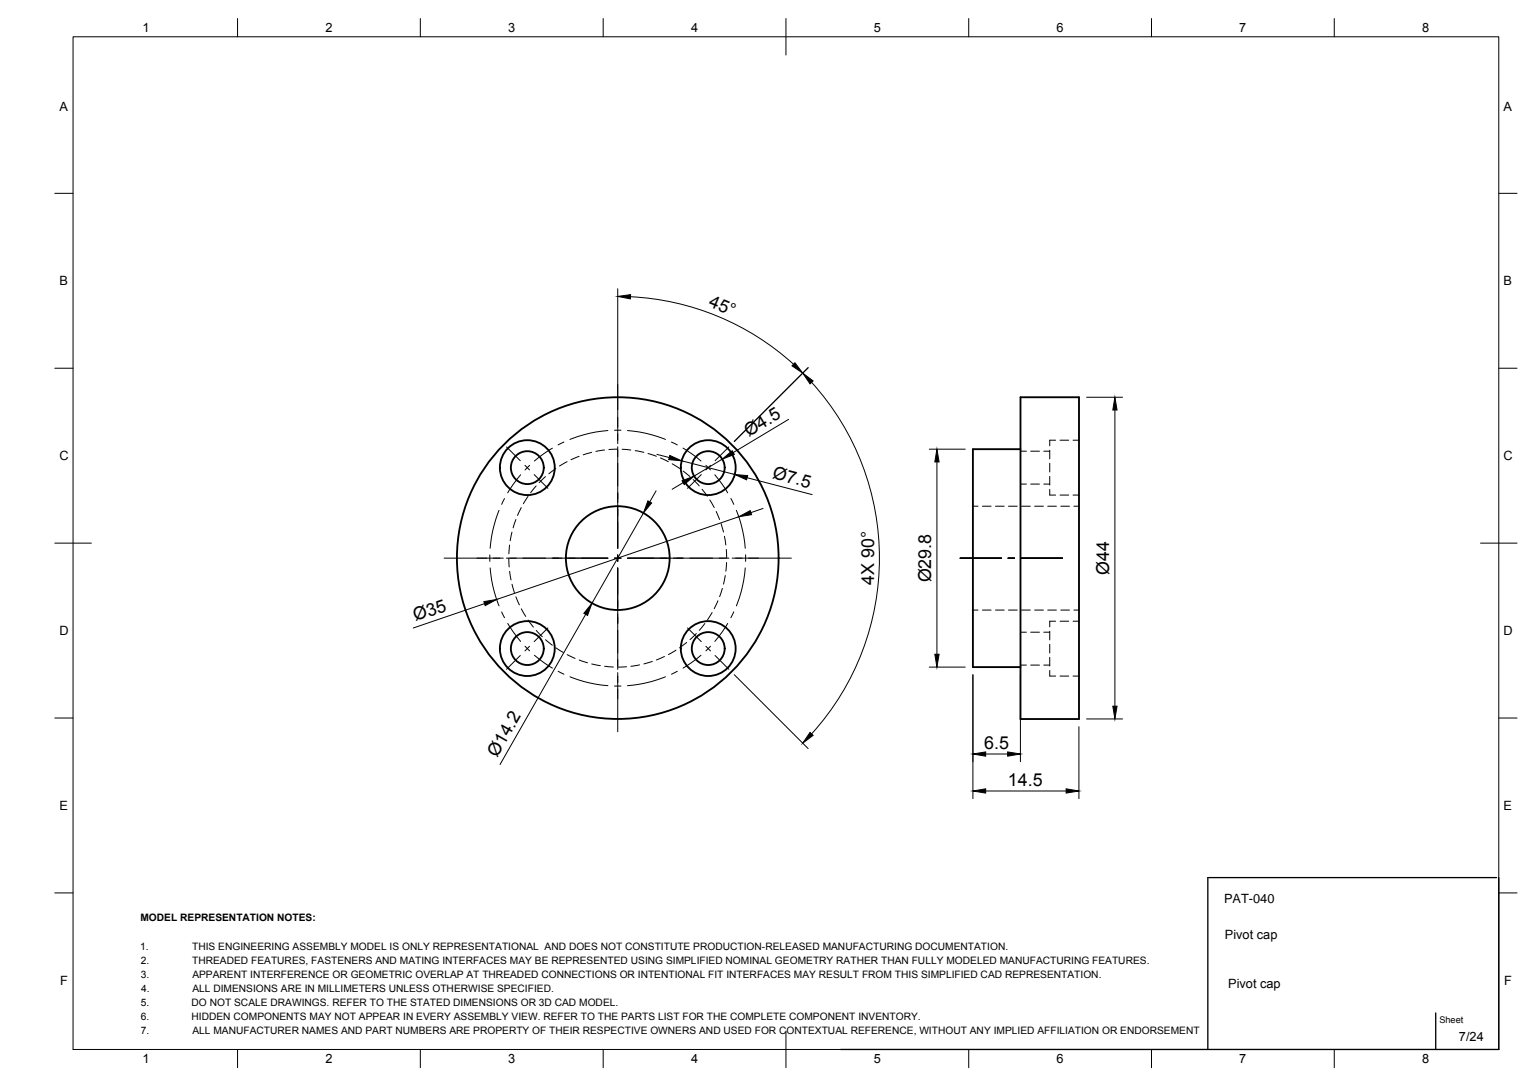
ISO-10303-21;
HEADER;
/* Generated by software containing ST-Developer
 * from STEP Tools, Inc. (www.steptools.com) 
 */

FILE_DESCRIPTION(
/* description */ ('Four-bar tabletop demonstrator'),
/* implementation_level */ '2;1');

FILE_NAME(
/* name */ 'Pivot cap.step',
/* time_stamp */ '2026-10-29T17:05:23-07:00',
/* author */ (''),
/* organization */ (''),
/* preprocessor_version */ 'ST-DEVELOPER v20.2',
/* originating_system */ 'Autodesk Translation Framework v15.17.0.0',
/* authorisation */ '');

FILE_SCHEMA (('AUTOMOTIVE_DESIGN { 1 0 10303 214 3 1 1 }'));
ENDSEC;

DATA;
#10=MECHANICAL_DESIGN_GEOMETRIC_PRESENTATION_REPRESENTATION('',(#354),#6705);
#316=SHAPE_REPRESENTATION_RELATIONSHIP('SRR','None',#6825,#331);
#331=ADVANCED_BREP_SHAPE_REPRESENTATION('',(#376),#6698);
#354=STYLED_ITEM('',(#6975),#376);
#376=MANIFOLD_SOLID_BREP('Body1',#3399);
#435=FACE_BOUND('',#954,.T.);
#436=FACE_BOUND('',#957,.T.);
#437=FACE_BOUND('',#960,.T.);
#438=FACE_BOUND('',#963,.T.);
#439=FACE_BOUND('',#970,.T.);
#440=FACE_BOUND('',#974,.T.);
#441=FACE_BOUND('',#975,.T.);
#442=FACE_BOUND('',#976,.T.);
#443=FACE_BOUND('',#977,.T.);
#444=FACE_BOUND('',#978,.T.);
#445=FACE_BOUND('',#980,.T.);
#446=FACE_BOUND('',#981,.T.);
#447=FACE_BOUND('',#982,.T.);
#448=FACE_BOUND('',#983,.T.);
#449=FACE_BOUND('',#984,.T.);
#521=PLANE('',#3885);
#522=PLANE('',#3890);
#523=PLANE('',#3895);
#524=PLANE('',#3900);
#525=PLANE('',#3913);
#526=PLANE('',#3920);
#527=PLANE('',#3921);
#695=FACE_OUTER_BOUND('',#952,.T.);
#696=FACE_OUTER_BOUND('',#953,.T.);
#697=FACE_OUTER_BOUND('',#955,.T.);
#698=FACE_OUTER_BOUND('',#956,.T.);
#699=FACE_OUTER_BOUND('',#958,.T.);
#700=FACE_OUTER_BOUND('',#959,.T.);
#701=FACE_OUTER_BOUND('',#961,.T.);
#702=FACE_OUTER_BOUND('',#962,.T.);
#703=FACE_OUTER_BOUND('',#964,.T.);
#704=FACE_OUTER_BOUND('',#965,.T.);
#705=FACE_OUTER_BOUND('',#966,.T.);
#706=FACE_OUTER_BOUND('',#967,.T.);
#707=FACE_OUTER_BOUND('',#968,.T.);
#708=FACE_OUTER_BOUND('',#969,.T.);
#709=FACE_OUTER_BOUND('',#971,.T.);
#710=FACE_OUTER_BOUND('',#972,.T.);
#711=FACE_OUTER_BOUND('',#973,.T.);
#712=FACE_OUTER_BOUND('',#979,.T.);
#952=EDGE_LOOP('',(#2840,#2841,#2842,#2843));
#953=EDGE_LOOP('',(#2844));
#954=EDGE_LOOP('',(#2845));
#955=EDGE_LOOP('',(#2846,#2847,#2848,#2849));
#956=EDGE_LOOP('',(#2850));
#957=EDGE_LOOP('',(#2851));
#958=EDGE_LOOP('',(#2852,#2853,#2854,#2855));
#959=EDGE_LOOP('',(#2856));
#960=EDGE_LOOP('',(#2857));
#961=EDGE_LOOP('',(#2858,#2859,#2860,#2861));
#962=EDGE_LOOP('',(#2862));
#963=EDGE_LOOP('',(#2863));
#964=EDGE_LOOP('',(#2864,#2865,#2866,#2867));
#965=EDGE_LOOP('',(#2868,#2869,#2870,#2871));
#966=EDGE_LOOP('',(#2872,#2873,#2874,#2875));
#967=EDGE_LOOP('',(#2876,#2877,#2878,#2879));
#968=EDGE_LOOP('',(#2880,#2881,#2882,#2883));
#969=EDGE_LOOP('',(#2884));
#970=EDGE_LOOP('',(#2885));
#971=EDGE_LOOP('',(#2886,#2887,#2888,#2889));
#972=EDGE_LOOP('',(#2890,#2891,#2892,#2893));
#973=EDGE_LOOP('',(#2894));
#974=EDGE_LOOP('',(#2895));
#975=EDGE_LOOP('',(#2896));
#976=EDGE_LOOP('',(#2897));
#977=EDGE_LOOP('',(#2898));
#978=EDGE_LOOP('',(#2899));
#979=EDGE_LOOP('',(#2900));
#980=EDGE_LOOP('',(#2901));
#981=EDGE_LOOP('',(#2902));
#982=EDGE_LOOP('',(#2903));
#983=EDGE_LOOP('',(#2904));
#984=EDGE_LOOP('',(#2905));
#1146=LINE('',#6256,#1316);
#1147=LINE('',#6265,#1317);
#1148=LINE('',#6274,#1318);
#1149=LINE('',#6283,#1319);
#1150=LINE('',#6291,#1320);
#1151=LINE('',#6295,#1321);
#1152=LINE('',#6299,#1322);
#1153=LINE('',#6303,#1323);
#1154=LINE('',#6308,#1324);
#1155=LINE('',#6316,#1325);
#1156=LINE('',#6321,#1326);
#1316=VECTOR('',#4787,0.375);
#1317=VECTOR('',#4798,0.375);
#1318=VECTOR('',#4809,0.375);
#1319=VECTOR('',#4820,0.375);
#1320=VECTOR('',#4831,0.225);
#1321=VECTOR('',#4836,0.225);
#1322=VECTOR('',#4841,0.225);
#1323=VECTOR('',#4846,0.225);
#1324=VECTOR('',#4851,1.49);
#1325=VECTOR('',#4862,0.71);
#1326=VECTOR('',#4867,2.2);
#1546=CIRCLE('',#3883,0.375);
#1547=CIRCLE('',#3884,0.375);
#1548=CIRCLE('',#3886,0.225);
#1549=CIRCLE('',#3888,0.375);
#1550=CIRCLE('',#3889,0.375);
#1551=CIRCLE('',#3891,0.225);
#1552=CIRCLE('',#3893,0.375);
#1553=CIRCLE('',#3894,0.375);
#1554=CIRCLE('',#3896,0.225);
#1555=CIRCLE('',#3898,0.375);
#1556=CIRCLE('',#3899,0.375);
#1557=CIRCLE('',#3901,0.225);
#1558=CIRCLE('',#3903,0.225);
#1559=CIRCLE('',#3905,0.225);
#1560=CIRCLE('',#3907,0.225);
#1561=CIRCLE('',#3909,0.225);
#1562=CIRCLE('',#3911,1.49);
#1563=CIRCLE('',#3912,1.49);
#1564=CIRCLE('',#3914,0.71);
#1565=CIRCLE('',#3916,0.71);
#1566=CIRCLE('',#3918,2.2);
#1567=CIRCLE('',#3919,2.2);
#1793=VERTEX_POINT('',#6253);
#1794=VERTEX_POINT('',#6255);
#1795=VERTEX_POINT('',#6259);
#1796=VERTEX_POINT('',#6262);
#1797=VERTEX_POINT('',#6264);
#1798=VERTEX_POINT('',#6268);
#1799=VERTEX_POINT('',#6271);
#1800=VERTEX_POINT('',#6273);
#1801=VERTEX_POINT('',#6277);
#1802=VERTEX_POINT('',#6280);
#1803=VERTEX_POINT('',#6282);
#1804=VERTEX_POINT('',#6286);
#1805=VERTEX_POINT('',#6289);
#1806=VERTEX_POINT('',#6293);
#1807=VERTEX_POINT('',#6297);
#1808=VERTEX_POINT('',#6301);
#1809=VERTEX_POINT('',#6305);
#1810=VERTEX_POINT('',#6307);
#1811=VERTEX_POINT('',#6311);
#1812=VERTEX_POINT('',#6314);
#1813=VERTEX_POINT('',#6318);
#1814=VERTEX_POINT('',#6320);
#2156=EDGE_CURVE('',#1793,#1793,#1546,.T.);
#2157=EDGE_CURVE('',#1793,#1794,#1146,.T.);
#2158=EDGE_CURVE('',#1794,#1794,#1547,.T.);
#2159=EDGE_CURVE('',#1795,#1795,#1548,.T.);
#2160=EDGE_CURVE('',#1796,#1796,#1549,.T.);
#2161=EDGE_CURVE('',#1796,#1797,#1147,.T.);
#2162=EDGE_CURVE('',#1797,#1797,#1550,.T.);
#2163=EDGE_CURVE('',#1798,#1798,#1551,.T.);
#2164=EDGE_CURVE('',#1799,#1799,#1552,.T.);
#2165=EDGE_CURVE('',#1799,#1800,#1148,.T.);
#2166=EDGE_CURVE('',#1800,#1800,#1553,.T.);
#2167=EDGE_CURVE('',#1801,#1801,#1554,.T.);
#2168=EDGE_CURVE('',#1802,#1802,#1555,.T.);
#2169=EDGE_CURVE('',#1802,#1803,#1149,.T.);
#2170=EDGE_CURVE('',#1803,#1803,#1556,.T.);
#2171=EDGE_CURVE('',#1804,#1804,#1557,.T.);
#2172=EDGE_CURVE('',#1805,#1805,#1558,.T.);
#2173=EDGE_CURVE('',#1805,#1795,#1150,.T.);
#2174=EDGE_CURVE('',#1806,#1806,#1559,.T.);
#2175=EDGE_CURVE('',#1806,#1798,#1151,.T.);
#2176=EDGE_CURVE('',#1807,#1807,#1560,.T.);
#2177=EDGE_CURVE('',#1807,#1801,#1152,.T.);
#2178=EDGE_CURVE('',#1808,#1808,#1561,.T.);
#2179=EDGE_CURVE('',#1808,#1804,#1153,.T.);
#2180=EDGE_CURVE('',#1809,#1809,#1562,.T.);
#2181=EDGE_CURVE('',#1809,#1810,#1154,.T.);
#2182=EDGE_CURVE('',#1810,#1810,#1563,.T.);
#2183=EDGE_CURVE('',#1811,#1811,#1564,.T.);
#2184=EDGE_CURVE('',#1812,#1812,#1565,.T.);
#2185=EDGE_CURVE('',#1812,#1811,#1155,.T.);
#2186=EDGE_CURVE('',#1813,#1813,#1566,.T.);
#2187=EDGE_CURVE('',#1813,#1814,#1156,.T.);
#2188=EDGE_CURVE('',#1814,#1814,#1567,.T.);
#2840=ORIENTED_EDGE('',*,*,#2156,.F.);
#2841=ORIENTED_EDGE('',*,*,#2157,.T.);
#2842=ORIENTED_EDGE('',*,*,#2158,.F.);
#2843=ORIENTED_EDGE('',*,*,#2157,.F.);
#2844=ORIENTED_EDGE('',*,*,#2156,.T.);
#2845=ORIENTED_EDGE('',*,*,#2159,.F.);
#2846=ORIENTED_EDGE('',*,*,#2160,.F.);
#2847=ORIENTED_EDGE('',*,*,#2161,.T.);
#2848=ORIENTED_EDGE('',*,*,#2162,.F.);
#2849=ORIENTED_EDGE('',*,*,#2161,.F.);
#2850=ORIENTED_EDGE('',*,*,#2160,.T.);
#2851=ORIENTED_EDGE('',*,*,#2163,.F.);
#2852=ORIENTED_EDGE('',*,*,#2164,.F.);
#2853=ORIENTED_EDGE('',*,*,#2165,.T.);
#2854=ORIENTED_EDGE('',*,*,#2166,.F.);
#2855=ORIENTED_EDGE('',*,*,#2165,.F.);
#2856=ORIENTED_EDGE('',*,*,#2164,.T.);
#2857=ORIENTED_EDGE('',*,*,#2167,.F.);
#2858=ORIENTED_EDGE('',*,*,#2168,.F.);
#2859=ORIENTED_EDGE('',*,*,#2169,.T.);
#2860=ORIENTED_EDGE('',*,*,#2170,.F.);
#2861=ORIENTED_EDGE('',*,*,#2169,.F.);
#2862=ORIENTED_EDGE('',*,*,#2168,.T.);
#2863=ORIENTED_EDGE('',*,*,#2171,.F.);
#2864=ORIENTED_EDGE('',*,*,#2172,.F.);
#2865=ORIENTED_EDGE('',*,*,#2173,.T.);
#2866=ORIENTED_EDGE('',*,*,#2159,.T.);
#2867=ORIENTED_EDGE('',*,*,#2173,.F.);
#2868=ORIENTED_EDGE('',*,*,#2174,.F.);
#2869=ORIENTED_EDGE('',*,*,#2175,.T.);
#2870=ORIENTED_EDGE('',*,*,#2163,.T.);
#2871=ORIENTED_EDGE('',*,*,#2175,.F.);
#2872=ORIENTED_EDGE('',*,*,#2176,.F.);
#2873=ORIENTED_EDGE('',*,*,#2177,.T.);
#2874=ORIENTED_EDGE('',*,*,#2167,.T.);
#2875=ORIENTED_EDGE('',*,*,#2177,.F.);
#2876=ORIENTED_EDGE('',*,*,#2178,.F.);
#2877=ORIENTED_EDGE('',*,*,#2179,.T.);
#2878=ORIENTED_EDGE('',*,*,#2171,.T.);
#2879=ORIENTED_EDGE('',*,*,#2179,.F.);
#2880=ORIENTED_EDGE('',*,*,#2180,.F.);
#2881=ORIENTED_EDGE('',*,*,#2181,.T.);
#2882=ORIENTED_EDGE('',*,*,#2182,.T.);
#2883=ORIENTED_EDGE('',*,*,#2181,.F.);
#2884=ORIENTED_EDGE('',*,*,#2182,.F.);
#2885=ORIENTED_EDGE('',*,*,#2183,.F.);
#2886=ORIENTED_EDGE('',*,*,#2184,.F.);
#2887=ORIENTED_EDGE('',*,*,#2185,.T.);
#2888=ORIENTED_EDGE('',*,*,#2183,.T.);
#2889=ORIENTED_EDGE('',*,*,#2185,.F.);
#2890=ORIENTED_EDGE('',*,*,#2186,.F.);
#2891=ORIENTED_EDGE('',*,*,#2187,.T.);
#2892=ORIENTED_EDGE('',*,*,#2188,.T.);
#2893=ORIENTED_EDGE('',*,*,#2187,.F.);
#2894=ORIENTED_EDGE('',*,*,#2186,.T.);
#2895=ORIENTED_EDGE('',*,*,#2184,.T.);
#2896=ORIENTED_EDGE('',*,*,#2170,.T.);
#2897=ORIENTED_EDGE('',*,*,#2166,.T.);
#2898=ORIENTED_EDGE('',*,*,#2162,.T.);
#2899=ORIENTED_EDGE('',*,*,#2158,.T.);
#2900=ORIENTED_EDGE('',*,*,#2188,.F.);
#2901=ORIENTED_EDGE('',*,*,#2180,.T.);
#2902=ORIENTED_EDGE('',*,*,#2178,.T.);
#2903=ORIENTED_EDGE('',*,*,#2176,.T.);
#2904=ORIENTED_EDGE('',*,*,#2174,.T.);
#2905=ORIENTED_EDGE('',*,*,#2172,.T.);
#3153=CYLINDRICAL_SURFACE('',#3882,0.375);
#3154=CYLINDRICAL_SURFACE('',#3887,0.375);
#3155=CYLINDRICAL_SURFACE('',#3892,0.375);
#3156=CYLINDRICAL_SURFACE('',#3897,0.375);
#3157=CYLINDRICAL_SURFACE('',#3902,0.225);
#3158=CYLINDRICAL_SURFACE('',#3904,0.225);
#3159=CYLINDRICAL_SURFACE('',#3906,0.225);
#3160=CYLINDRICAL_SURFACE('',#3908,0.225);
#3161=CYLINDRICAL_SURFACE('',#3910,1.49);
#3162=CYLINDRICAL_SURFACE('',#3915,0.71);
#3163=CYLINDRICAL_SURFACE('',#3917,2.2);
#3311=ADVANCED_FACE('',(#695),#3153,.F.);
#3312=ADVANCED_FACE('',(#696,#435),#521,.T.);
#3313=ADVANCED_FACE('',(#697),#3154,.F.);
#3314=ADVANCED_FACE('',(#698,#436),#522,.T.);
#3315=ADVANCED_FACE('',(#699),#3155,.F.);
#3316=ADVANCED_FACE('',(#700,#437),#523,.T.);
#3317=ADVANCED_FACE('',(#701),#3156,.F.);
#3318=ADVANCED_FACE('',(#702,#438),#524,.T.);
#3319=ADVANCED_FACE('',(#703),#3157,.F.);
#3320=ADVANCED_FACE('',(#704),#3158,.F.);
#3321=ADVANCED_FACE('',(#705),#3159,.F.);
#3322=ADVANCED_FACE('',(#706),#3160,.F.);
#3323=ADVANCED_FACE('',(#707),#3161,.T.);
#3324=ADVANCED_FACE('',(#708,#439),#525,.F.);
#3325=ADVANCED_FACE('',(#709),#3162,.F.);
#3326=ADVANCED_FACE('',(#710),#3163,.T.);
#3327=ADVANCED_FACE('',(#711,#440,#441,#442,#443,#444),#526,.T.);
#3328=ADVANCED_FACE('',(#712,#445,#446,#447,#448,#449),#527,.F.);
#3399=CLOSED_SHELL('',(#3311,#3312,#3313,#3314,#3315,#3316,#3317,#3318,
#3319,#3320,#3321,#3322,#3323,#3324,#3325,#3326,#3327,#3328));
#3881=AXIS2_PLACEMENT_3D('',#6251,#4781,#4782);
#3882=AXIS2_PLACEMENT_3D('',#6252,#4783,#4784);
#3883=AXIS2_PLACEMENT_3D('',#6254,#4785,#4786);
#3884=AXIS2_PLACEMENT_3D('',#6257,#4788,#4789);
#3885=AXIS2_PLACEMENT_3D('',#6258,#4790,#4791);
#3886=AXIS2_PLACEMENT_3D('',#6260,#4792,#4793);
#3887=AXIS2_PLACEMENT_3D('',#6261,#4794,#4795);
#3888=AXIS2_PLACEMENT_3D('',#6263,#4796,#4797);
#3889=AXIS2_PLACEMENT_3D('',#6266,#4799,#4800);
#3890=AXIS2_PLACEMENT_3D('',#6267,#4801,#4802);
#3891=AXIS2_PLACEMENT_3D('',#6269,#4803,#4804);
#3892=AXIS2_PLACEMENT_3D('',#6270,#4805,#4806);
#3893=AXIS2_PLACEMENT_3D('',#6272,#4807,#4808);
#3894=AXIS2_PLACEMENT_3D('',#6275,#4810,#4811);
#3895=AXIS2_PLACEMENT_3D('',#6276,#4812,#4813);
#3896=AXIS2_PLACEMENT_3D('',#6278,#4814,#4815);
#3897=AXIS2_PLACEMENT_3D('',#6279,#4816,#4817);
#3898=AXIS2_PLACEMENT_3D('',#6281,#4818,#4819);
#3899=AXIS2_PLACEMENT_3D('',#6284,#4821,#4822);
#3900=AXIS2_PLACEMENT_3D('',#6285,#4823,#4824);
#3901=AXIS2_PLACEMENT_3D('',#6287,#4825,#4826);
#3902=AXIS2_PLACEMENT_3D('',#6288,#4827,#4828);
#3903=AXIS2_PLACEMENT_3D('',#6290,#4829,#4830);
#3904=AXIS2_PLACEMENT_3D('',#6292,#4832,#4833);
#3905=AXIS2_PLACEMENT_3D('',#6294,#4834,#4835);
#3906=AXIS2_PLACEMENT_3D('',#6296,#4837,#4838);
#3907=AXIS2_PLACEMENT_3D('',#6298,#4839,#4840);
#3908=AXIS2_PLACEMENT_3D('',#6300,#4842,#4843);
#3909=AXIS2_PLACEMENT_3D('',#6302,#4844,#4845);
#3910=AXIS2_PLACEMENT_3D('',#6304,#4847,#4848);
#3911=AXIS2_PLACEMENT_3D('',#6306,#4849,#4850);
#3912=AXIS2_PLACEMENT_3D('',#6309,#4852,#4853);
#3913=AXIS2_PLACEMENT_3D('',#6310,#4854,#4855);
#3914=AXIS2_PLACEMENT_3D('',#6312,#4856,#4857);
#3915=AXIS2_PLACEMENT_3D('',#6313,#4858,#4859);
#3916=AXIS2_PLACEMENT_3D('',#6315,#4860,#4861);
#3917=AXIS2_PLACEMENT_3D('',#6317,#4863,#4864);
#3918=AXIS2_PLACEMENT_3D('',#6319,#4865,#4866);
#3919=AXIS2_PLACEMENT_3D('',#6322,#4868,#4869);
#3920=AXIS2_PLACEMENT_3D('',#6323,#4870,#4871);
#3921=AXIS2_PLACEMENT_3D('',#6324,#4872,#4873);
#4781=DIRECTION('axis',(0.,0.,1.));
#4782=DIRECTION('refdir',(1.,0.,0.));
#4783=DIRECTION('center_axis',(0.,0.,1.));
#4784=DIRECTION('ref_axis',(1.,0.,0.));
#4785=DIRECTION('center_axis',(0.,0.,1.));
#4786=DIRECTION('ref_axis',(1.,0.,0.));
#4787=DIRECTION('',(0.,0.,1.));
#4788=DIRECTION('center_axis',(0.,0.,-1.));
#4789=DIRECTION('ref_axis',(1.,0.,0.));
#4790=DIRECTION('center_axis',(0.,0.,1.));
#4791=DIRECTION('ref_axis',(1.,0.,0.));
#4792=DIRECTION('center_axis',(0.,0.,1.));
#4793=DIRECTION('ref_axis',(1.,0.,0.));
#4794=DIRECTION('center_axis',(0.,0.,1.));
#4795=DIRECTION('ref_axis',(1.,0.,0.));
#4796=DIRECTION('center_axis',(0.,0.,1.));
#4797=DIRECTION('ref_axis',(1.,0.,0.));
#4798=DIRECTION('',(0.,0.,1.));
#4799=DIRECTION('center_axis',(0.,0.,-1.));
#4800=DIRECTION('ref_axis',(1.,0.,0.));
#4801=DIRECTION('center_axis',(0.,0.,1.));
#4802=DIRECTION('ref_axis',(1.,0.,0.));
#4803=DIRECTION('center_axis',(0.,0.,1.));
#4804=DIRECTION('ref_axis',(1.,0.,0.));
#4805=DIRECTION('center_axis',(0.,0.,1.));
#4806=DIRECTION('ref_axis',(1.,0.,0.));
#4807=DIRECTION('center_axis',(0.,0.,1.));
#4808=DIRECTION('ref_axis',(1.,0.,0.));
#4809=DIRECTION('',(0.,0.,1.));
#4810=DIRECTION('center_axis',(0.,0.,-1.));
#4811=DIRECTION('ref_axis',(1.,0.,0.));
#4812=DIRECTION('center_axis',(0.,0.,1.));
#4813=DIRECTION('ref_axis',(1.,0.,0.));
#4814=DIRECTION('center_axis',(0.,0.,1.));
#4815=DIRECTION('ref_axis',(1.,0.,0.));
#4816=DIRECTION('center_axis',(0.,0.,1.));
#4817=DIRECTION('ref_axis',(1.,0.,0.));
#4818=DIRECTION('center_axis',(0.,0.,1.));
#4819=DIRECTION('ref_axis',(1.,0.,0.));
#4820=DIRECTION('',(0.,0.,1.));
#4821=DIRECTION('center_axis',(0.,0.,-1.));
#4822=DIRECTION('ref_axis',(1.,0.,0.));
#4823=DIRECTION('center_axis',(0.,0.,1.));
#4824=DIRECTION('ref_axis',(1.,0.,0.));
#4825=DIRECTION('center_axis',(0.,0.,1.));
#4826=DIRECTION('ref_axis',(1.,0.,0.));
#4827=DIRECTION('center_axis',(0.,0.,1.));
#4828=DIRECTION('ref_axis',(1.,0.,0.));
#4829=DIRECTION('center_axis',(0.,0.,1.));
#4830=DIRECTION('ref_axis',(1.,0.,0.));
#4831=DIRECTION('',(0.,0.,1.));
#4832=DIRECTION('center_axis',(0.,0.,1.));
#4833=DIRECTION('ref_axis',(1.,0.,0.));
#4834=DIRECTION('center_axis',(0.,0.,1.));
#4835=DIRECTION('ref_axis',(1.,0.,0.));
#4836=DIRECTION('',(0.,0.,1.));
#4837=DIRECTION('center_axis',(0.,0.,1.));
#4838=DIRECTION('ref_axis',(1.,0.,0.));
#4839=DIRECTION('center_axis',(0.,0.,1.));
#4840=DIRECTION('ref_axis',(1.,0.,0.));
#4841=DIRECTION('',(0.,0.,1.));
#4842=DIRECTION('center_axis',(0.,0.,1.));
#4843=DIRECTION('ref_axis',(1.,0.,0.));
#4844=DIRECTION('center_axis',(0.,0.,1.));
#4845=DIRECTION('ref_axis',(1.,0.,0.));
#4846=DIRECTION('',(0.,0.,1.));
#4847=DIRECTION('center_axis',(0.,0.,1.));
#4848=DIRECTION('ref_axis',(1.,0.,0.));
#4849=DIRECTION('center_axis',(0.,0.,1.));
#4850=DIRECTION('ref_axis',(1.,0.,0.));
#4851=DIRECTION('',(0.,0.,-1.));
#4852=DIRECTION('center_axis',(0.,0.,1.));
#4853=DIRECTION('ref_axis',(1.,0.,0.));
#4854=DIRECTION('center_axis',(0.,0.,1.));
#4855=DIRECTION('ref_axis',(1.,0.,0.));
#4856=DIRECTION('center_axis',(0.,0.,-1.));
#4857=DIRECTION('ref_axis',(1.,0.,0.));
#4858=DIRECTION('center_axis',(0.,0.,1.));
#4859=DIRECTION('ref_axis',(1.,0.,0.));
#4860=DIRECTION('center_axis',(0.,0.,-1.));
#4861=DIRECTION('ref_axis',(1.,0.,0.));
#4862=DIRECTION('',(0.,0.,-1.));
#4863=DIRECTION('center_axis',(0.,0.,1.));
#4864=DIRECTION('ref_axis',(1.,0.,0.));
#4865=DIRECTION('center_axis',(0.,0.,1.));
#4866=DIRECTION('ref_axis',(1.,0.,0.));
#4867=DIRECTION('',(0.,0.,-1.));
#4868=DIRECTION('center_axis',(0.,0.,1.));
#4869=DIRECTION('ref_axis',(1.,0.,0.));
#4870=DIRECTION('center_axis',(0.,0.,1.));
#4871=DIRECTION('ref_axis',(1.,0.,0.));
#4872=DIRECTION('center_axis',(0.,0.,1.));
#4873=DIRECTION('ref_axis',(1.,0.,0.));
#6251=CARTESIAN_POINT('',(0.,0.,0.));
#6252=CARTESIAN_POINT('Origin',(-1.23743686707646,-1.23743686707646,4.));
#6253=CARTESIAN_POINT('',(-1.61243686707646,-1.23743686707646,4.));
#6254=CARTESIAN_POINT('Origin',(-1.23743686707646,-1.23743686707646,4.));
#6255=CARTESIAN_POINT('',(-1.61243686707646,-1.23743686707646,4.4));
#6256=CARTESIAN_POINT('',(-1.61243686707646,-1.23743686707646,4.));
#6257=CARTESIAN_POINT('Origin',(-1.23743686707646,-1.23743686707646,4.4));
#6258=CARTESIAN_POINT('Origin',(-1.23743686707646,-1.23743686707646,4.));
#6259=CARTESIAN_POINT('',(-1.46243686707646,-1.23743686707646,4.));
#6260=CARTESIAN_POINT('Origin',(-1.23743686707646,-1.23743686707646,4.));
#6261=CARTESIAN_POINT('Origin',(-1.23743686707646,1.23743686707646,4.));
#6262=CARTESIAN_POINT('',(-1.61243686707646,1.23743686707646,4.));
#6263=CARTESIAN_POINT('Origin',(-1.23743686707646,1.23743686707646,4.));
#6264=CARTESIAN_POINT('',(-1.61243686707646,1.23743686707646,4.4));
#6265=CARTESIAN_POINT('',(-1.61243686707646,1.23743686707646,4.));
#6266=CARTESIAN_POINT('Origin',(-1.23743686707646,1.23743686707646,4.4));
#6267=CARTESIAN_POINT('Origin',(-1.23743686707646,1.23743686707646,4.));
#6268=CARTESIAN_POINT('',(-1.46243686707646,1.23743686707646,4.));
#6269=CARTESIAN_POINT('Origin',(-1.23743686707646,1.23743686707646,4.));
#6270=CARTESIAN_POINT('Origin',(1.23743686707646,1.23743686707646,4.));
#6271=CARTESIAN_POINT('',(0.862436867076458,1.23743686707646,4.));
#6272=CARTESIAN_POINT('Origin',(1.23743686707646,1.23743686707646,4.));
#6273=CARTESIAN_POINT('',(0.862436867076458,1.23743686707646,4.4));
#6274=CARTESIAN_POINT('',(0.862436867076458,1.23743686707646,4.));
#6275=CARTESIAN_POINT('Origin',(1.23743686707646,1.23743686707646,4.4));
#6276=CARTESIAN_POINT('Origin',(1.23743686707646,1.23743686707646,4.));
#6277=CARTESIAN_POINT('',(1.01243686707646,1.23743686707646,4.));
#6278=CARTESIAN_POINT('Origin',(1.23743686707646,1.23743686707646,4.));
#6279=CARTESIAN_POINT('Origin',(1.23743686707646,-1.23743686707646,4.));
#6280=CARTESIAN_POINT('',(0.862436867076458,-1.23743686707646,4.));
#6281=CARTESIAN_POINT('Origin',(1.23743686707646,-1.23743686707646,4.));
#6282=CARTESIAN_POINT('',(0.862436867076458,-1.23743686707646,4.4));
#6283=CARTESIAN_POINT('',(0.862436867076458,-1.23743686707646,4.));
#6284=CARTESIAN_POINT('Origin',(1.23743686707646,-1.23743686707646,4.4));
#6285=CARTESIAN_POINT('Origin',(1.23743686707646,-1.23743686707646,4.));
#6286=CARTESIAN_POINT('',(1.01243686707646,-1.23743686707646,4.));
#6287=CARTESIAN_POINT('Origin',(1.23743686707646,-1.23743686707646,4.));
#6288=CARTESIAN_POINT('Origin',(-1.23743686707646,-1.23743686707646,3.5));
#6289=CARTESIAN_POINT('',(-1.46243686707646,-1.23743686707646,3.6));
#6290=CARTESIAN_POINT('Origin',(-1.23743686707646,-1.23743686707646,3.6));
#6291=CARTESIAN_POINT('',(-1.46243686707646,-1.23743686707646,3.5));
#6292=CARTESIAN_POINT('Origin',(-1.23743686707646,1.23743686707646,3.5));
#6293=CARTESIAN_POINT('',(-1.46243686707646,1.23743686707646,3.6));
#6294=CARTESIAN_POINT('Origin',(-1.23743686707646,1.23743686707646,3.6));
#6295=CARTESIAN_POINT('',(-1.46243686707646,1.23743686707646,3.5));
#6296=CARTESIAN_POINT('Origin',(1.23743686707646,1.23743686707646,3.5));
#6297=CARTESIAN_POINT('',(1.01243686707646,1.23743686707646,3.6));
#6298=CARTESIAN_POINT('Origin',(1.23743686707646,1.23743686707646,3.6));
#6299=CARTESIAN_POINT('',(1.01243686707646,1.23743686707646,3.5));
#6300=CARTESIAN_POINT('Origin',(1.23743686707646,-1.23743686707646,3.5));
#6301=CARTESIAN_POINT('',(1.01243686707646,-1.23743686707646,3.6));
#6302=CARTESIAN_POINT('Origin',(1.23743686707646,-1.23743686707646,3.6));
#6303=CARTESIAN_POINT('',(1.01243686707646,-1.23743686707646,3.5));
#6304=CARTESIAN_POINT('Origin',(0.,0.,2.95));
#6305=CARTESIAN_POINT('',(-1.49,-1.82472373072956E-16,3.6));
#6306=CARTESIAN_POINT('Origin',(0.,0.,3.6));
#6307=CARTESIAN_POINT('',(-1.49,-1.82472373072956E-16,2.95));
#6308=CARTESIAN_POINT('',(-1.49,-1.82472373072956E-16,2.95));
#6309=CARTESIAN_POINT('Origin',(0.,0.,2.95));
#6310=CARTESIAN_POINT('Origin',(0.,0.,2.95));
#6311=CARTESIAN_POINT('',(-0.71,-8.69499227394621E-17,2.95));
#6312=CARTESIAN_POINT('Origin',(0.,0.,2.95));
#6313=CARTESIAN_POINT('Origin',(0.,0.,3.6));
#6314=CARTESIAN_POINT('',(-0.71,-8.69499227394621E-17,4.4));
#6315=CARTESIAN_POINT('Origin',(0.,0.,4.4));
#6316=CARTESIAN_POINT('',(-0.71,-8.69499227394621E-17,3.6));
#6317=CARTESIAN_POINT('Origin',(0.,0.,3.6));
#6318=CARTESIAN_POINT('',(-2.2,-2.69422295812418E-16,4.4));
#6319=CARTESIAN_POINT('Origin',(0.,0.,4.4));
#6320=CARTESIAN_POINT('',(-2.2,-2.69422295812418E-16,3.6));
#6321=CARTESIAN_POINT('',(-2.2,-2.69422295812418E-16,3.6));
#6322=CARTESIAN_POINT('Origin',(0.,0.,3.6));
#6323=CARTESIAN_POINT('Origin',(0.,0.,4.4));
#6324=CARTESIAN_POINT('Origin',(0.,0.,3.6));
#6676=UNCERTAINTY_MEASURE_WITH_UNIT(LENGTH_MEASURE(0.001),#6706,
'DISTANCE_ACCURACY_VALUE',
'Maximum model space distance between geometric entities at asserted c
onnectivities');
#6683=UNCERTAINTY_MEASURE_WITH_UNIT(LENGTH_MEASURE(0.001),#6706,
'DISTANCE_ACCURACY_VALUE',
'Maximum model space distance between geometric entities at asserted c
onnectivities');
#6698=(
GEOMETRIC_REPRESENTATION_CONTEXT(3)
GLOBAL_UNCERTAINTY_ASSIGNED_CONTEXT((#6676))
GLOBAL_UNIT_ASSIGNED_CONTEXT((#6706,#6708,#6709))
REPRESENTATION_CONTEXT('','3D')
);
#6705=(
GEOMETRIC_REPRESENTATION_CONTEXT(3)
GLOBAL_UNCERTAINTY_ASSIGNED_CONTEXT((#6683))
GLOBAL_UNIT_ASSIGNED_CONTEXT((#6706,#6708,#6709))
REPRESENTATION_CONTEXT('','3D')
);
#6706=(
LENGTH_UNIT()
NAMED_UNIT(*)
SI_UNIT(.CENTI.,.METRE.)
);
#6708=(
NAMED_UNIT(*)
PLANE_ANGLE_UNIT()
SI_UNIT($,.RADIAN.)
);
#6709=(
NAMED_UNIT(*)
SI_UNIT($,.STERADIAN.)
SOLID_ANGLE_UNIT()
);
#6724=SHAPE_DEFINITION_REPRESENTATION(#6750,#6825);
#6750=PRODUCT_DEFINITION_SHAPE('',$,#6847);
#6825=SHAPE_REPRESENTATION('',(#3881),#6698);
#6832=PRODUCT_DEFINITION_CONTEXT('part definition',#6897,'design');
#6847=PRODUCT_DEFINITION('Pivot cap','Pivot cap',#6868,#6832);
#6868=PRODUCT_DEFINITION_FORMATION('',$,#6913);
#6897=APPLICATION_CONTEXT(
'Core Data for Automotive Mechanical Design Process');
#6898=PRODUCT_CONTEXT('part definition',#6897,'mechanical');
#6913=PRODUCT('Pivot cap','Pivot cap','Pivot cap',(#6898));
#6969=COLOUR_RGB('Light Blue',0.38,0.62,0.78);
#6970=FILL_AREA_STYLE_COLOUR('',#6969);
#6971=FILL_AREA_STYLE('',(#6970));
#6972=SURFACE_STYLE_FILL_AREA(#6971);
#6973=SURFACE_SIDE_STYLE('',(#6972));
#6974=SURFACE_STYLE_USAGE(.BOTH.,#6973);
#6975=PRESENTATION_STYLE_ASSIGNMENT((#6974));
ENDSEC;
END-ISO-10303-21;
